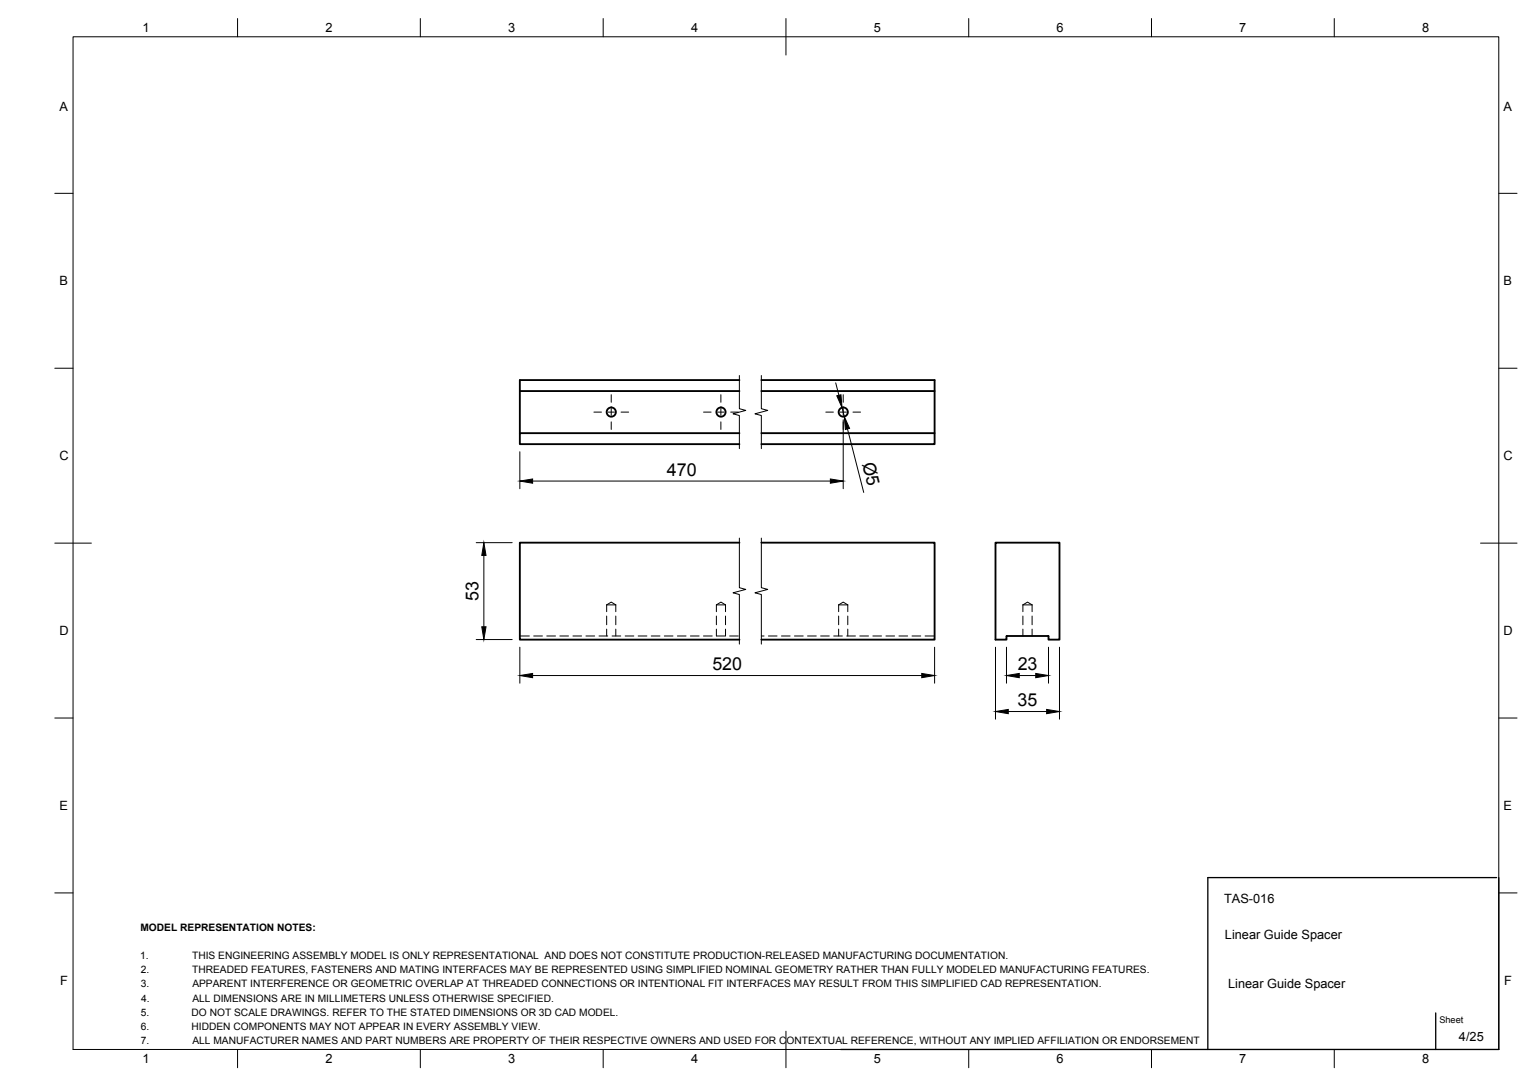
ISO-10303-21;
HEADER;
/* Generated by software containing ST-Developer
 * from STEP Tools, Inc. (www.steptools.com) 
 */

FILE_DESCRIPTION(
/* description */ ('STEP AP214'),
/* implementation_level */ '2;1');

FILE_NAME(
/* name */ 'Linear Guide Spacer.step',
/* time_stamp */ '2026-11-15T14:55:55-08:00',
/* author */ (''),
/* organization */ (''),
/* preprocessor_version */ 'ST-DEVELOPER v20.2',
/* originating_system */ 'Autodesk Translation Framework v15.17.0.0',
/* authorisation */ '');

FILE_SCHEMA (('AUTOMOTIVE_DESIGN { 1 0 10303 214 3 1 1 }'));
ENDSEC;

DATA;
#10=MECHANICAL_DESIGN_GEOMETRIC_PRESENTATION_REPRESENTATION('',(#953),#57079);
#891=SHAPE_REPRESENTATION_RELATIONSHIP('SRR','None',#57281,#920);
#920=ADVANCED_BREP_SHAPE_REPRESENTATION('',(#990),#57073);
#953=STYLED_ITEM('',(#57444),#990);
#990=MANIFOLD_SOLID_BREP('Body1',#24553);
#1318=FACE_BOUND('',#5120,.T.);
#1319=FACE_BOUND('',#5121,.T.);
#1320=FACE_BOUND('',#5122,.T.);
#1321=FACE_BOUND('',#5123,.T.);
#1322=FACE_BOUND('',#5124,.T.);
#1323=FACE_BOUND('',#5125,.T.);
#1324=FACE_BOUND('',#5126,.T.);
#1325=FACE_BOUND('',#5127,.T.);
#2021=PLANE('',#27222);
#2022=PLANE('',#27223);
#2023=PLANE('',#27226);
#2024=PLANE('',#27227);
#2025=PLANE('',#27230);
#2026=PLANE('',#27231);
#2027=PLANE('',#27232);
#2028=PLANE('',#27233);
#2029=PLANE('',#27234);
#2030=PLANE('',#27235);
#2141=CONICAL_SURFACE('',#27193,2.5,1.02974425867665);
#2142=CONICAL_SURFACE('',#27197,2.5,1.02974425867665);
#2143=CONICAL_SURFACE('',#27201,2.5,1.02974425867665);
#2144=CONICAL_SURFACE('',#27205,2.5,1.02974425867665);
#2145=CONICAL_SURFACE('',#27209,2.5,1.02974425867665);
#2146=CONICAL_SURFACE('',#27213,2.5,1.02974425867665);
#2147=CONICAL_SURFACE('',#27217,2.5,1.02974425867665);
#2148=CONICAL_SURFACE('',#27221,2.5,1.02974425867665);
#3402=FACE_OUTER_BOUND('',#5095,.T.);
#3403=FACE_OUTER_BOUND('',#5096,.T.);
#3404=FACE_OUTER_BOUND('',#5097,.T.);
#3405=FACE_OUTER_BOUND('',#5098,.T.);
#3406=FACE_OUTER_BOUND('',#5099,.T.);
#3407=FACE_OUTER_BOUND('',#5100,.T.);
#3408=FACE_OUTER_BOUND('',#5101,.T.);
#3409=FACE_OUTER_BOUND('',#5102,.T.);
#3410=FACE_OUTER_BOUND('',#5103,.T.);
#3411=FACE_OUTER_BOUND('',#5104,.T.);
#3412=FACE_OUTER_BOUND('',#5105,.T.);
#3413=FACE_OUTER_BOUND('',#5106,.T.);
#3414=FACE_OUTER_BOUND('',#5107,.T.);
#3415=FACE_OUTER_BOUND('',#5108,.T.);
#3416=FACE_OUTER_BOUND('',#5109,.T.);
#3417=FACE_OUTER_BOUND('',#5110,.T.);
#3418=FACE_OUTER_BOUND('',#5111,.T.);
#3419=FACE_OUTER_BOUND('',#5112,.T.);
#3420=FACE_OUTER_BOUND('',#5113,.T.);
#3421=FACE_OUTER_BOUND('',#5114,.T.);
#3422=FACE_OUTER_BOUND('',#5115,.T.);
#3423=FACE_OUTER_BOUND('',#5116,.T.);
#3424=FACE_OUTER_BOUND('',#5117,.T.);
#3425=FACE_OUTER_BOUND('',#5118,.T.);
#3426=FACE_OUTER_BOUND('',#5119,.T.);
#3427=FACE_OUTER_BOUND('',#5128,.T.);
#3428=FACE_OUTER_BOUND('',#5129,.T.);
#3429=FACE_OUTER_BOUND('',#5130,.T.);
#5095=EDGE_LOOP('',(#22196,#22197,#22198,#22199));
#5096=EDGE_LOOP('',(#22200,#22201,#22202));
#5097=EDGE_LOOP('',(#22203,#22204,#22205,#22206));
#5098=EDGE_LOOP('',(#22207,#22208,#22209));
#5099=EDGE_LOOP('',(#22210,#22211,#22212,#22213));
#5100=EDGE_LOOP('',(#22214,#22215,#22216));
#5101=EDGE_LOOP('',(#22217,#22218,#22219,#22220));
#5102=EDGE_LOOP('',(#22221,#22222,#22223));
#5103=EDGE_LOOP('',(#22224,#22225,#22226,#22227));
#5104=EDGE_LOOP('',(#22228,#22229,#22230));
#5105=EDGE_LOOP('',(#22231,#22232,#22233,#22234));
#5106=EDGE_LOOP('',(#22235,#22236,#22237));
#5107=EDGE_LOOP('',(#22238,#22239,#22240,#22241));
#5108=EDGE_LOOP('',(#22242,#22243,#22244));
#5109=EDGE_LOOP('',(#22245,#22246,#22247,#22248));
#5110=EDGE_LOOP('',(#22249,#22250,#22251));
#5111=EDGE_LOOP('',(#22252,#22253,#22254,#22255));
#5112=EDGE_LOOP('',(#22256,#22257,#22258,#22259,#22260,#22261,#22262,#22263,
#22264,#22265));
#5113=EDGE_LOOP('',(#22266,#22267,#22268,#22269));
#5114=EDGE_LOOP('',(#22270,#22271,#22272,#22273,#22274,#22275,#22276,#22277,
#22278,#22279));
#5115=EDGE_LOOP('',(#22280,#22281,#22282,#22283));
#5116=EDGE_LOOP('',(#22284,#22285,#22286,#22287));
#5117=EDGE_LOOP('',(#22288,#22289,#22290,#22291));
#5118=EDGE_LOOP('',(#22292,#22293,#22294,#22295));
#5119=EDGE_LOOP('',(#22296,#22297,#22298,#22299));
#5120=EDGE_LOOP('',(#22300));
#5121=EDGE_LOOP('',(#22301));
#5122=EDGE_LOOP('',(#22302));
#5123=EDGE_LOOP('',(#22303));
#5124=EDGE_LOOP('',(#22304));
#5125=EDGE_LOOP('',(#22305));
#5126=EDGE_LOOP('',(#22306));
#5127=EDGE_LOOP('',(#22307));
#5128=EDGE_LOOP('',(#22308,#22309,#22310,#22311));
#5129=EDGE_LOOP('',(#22312,#22313,#22314,#22315));
#5130=EDGE_LOOP('',(#22316,#22317,#22318,#22319));
#7032=LINE('',#56352,#8999);
#7033=LINE('',#56356,#9000);
#7034=LINE('',#56361,#9001);
#7035=LINE('',#56365,#9002);
#7036=LINE('',#56370,#9003);
#7037=LINE('',#56374,#9004);
#7038=LINE('',#56379,#9005);
#7039=LINE('',#56383,#9006);
#7040=LINE('',#56388,#9007);
#7041=LINE('',#56392,#9008);
#7042=LINE('',#56397,#9009);
#7043=LINE('',#56401,#9010);
#7044=LINE('',#56406,#9011);
#7045=LINE('',#56410,#9012);
#7046=LINE('',#56415,#9013);
#7047=LINE('',#56419,#9014);
#7048=LINE('',#56423,#9015);
#7049=LINE('',#56425,#9016);
#7050=LINE('',#56427,#9017);
#7051=LINE('',#56428,#9018);
#7052=LINE('',#56431,#9019);
#7053=LINE('',#56435,#9020);
#7054=LINE('',#56439,#9021);
#7055=LINE('',#56441,#9022);
#7056=LINE('',#56443,#9023);
#7057=LINE('',#56445,#9024);
#7058=LINE('',#56446,#9025);
#7059=LINE('',#56449,#9026);
#7060=LINE('',#56451,#9027);
#7061=LINE('',#56452,#9028);
#7062=LINE('',#56456,#9029);
#7063=LINE('',#56460,#9030);
#7064=LINE('',#56463,#9031);
#7065=LINE('',#56464,#9032);
#7066=LINE('',#56466,#9033);
#7067=LINE('',#56467,#9034);
#7068=LINE('',#56469,#9035);
#7069=LINE('',#56470,#9036);
#7070=LINE('',#56474,#9037);
#7071=LINE('',#56476,#9038);
#7072=LINE('',#56477,#9039);
#7073=LINE('',#56479,#9040);
#8999=VECTOR('',#33876,2.5);
#9000=VECTOR('',#33881,2.5);
#9001=VECTOR('',#33886,2.5);
#9002=VECTOR('',#33891,2.5);
#9003=VECTOR('',#33896,2.5);
#9004=VECTOR('',#33901,2.5);
#9005=VECTOR('',#33906,2.5);
#9006=VECTOR('',#33911,2.5);
#9007=VECTOR('',#33916,2.5);
#9008=VECTOR('',#33921,2.5);
#9009=VECTOR('',#33926,2.5);
#9010=VECTOR('',#33931,2.5);
#9011=VECTOR('',#33936,2.5);
#9012=VECTOR('',#33941,2.5);
#9013=VECTOR('',#33946,2.5);
#9014=VECTOR('',#33951,2.5);
#9015=VECTOR('',#33954,1000.);
#9016=VECTOR('',#33955,1000.);
#9017=VECTOR('',#33956,1000.);
#9018=VECTOR('',#33957,1000.);
#9019=VECTOR('',#33960,1000.);
#9020=VECTOR('',#33963,1000.);
#9021=VECTOR('',#33966,1000.);
#9022=VECTOR('',#33967,1000.);
#9023=VECTOR('',#33968,1000.);
#9024=VECTOR('',#33969,1000.);
#9025=VECTOR('',#33970,1000.);
#9026=VECTOR('',#33973,1000.);
#9027=VECTOR('',#33974,1000.);
#9028=VECTOR('',#33975,1000.);
#9029=VECTOR('',#33978,1000.);
#9030=VECTOR('',#33981,1000.);
#9031=VECTOR('',#33984,1000.);
#9032=VECTOR('',#33985,1000.);
#9033=VECTOR('',#33986,1000.);
#9034=VECTOR('',#33987,1000.);
#9035=VECTOR('',#33990,1000.);
#9036=VECTOR('',#33991,1000.);
#9037=VECTOR('',#33998,1000.);
#9038=VECTOR('',#34001,1000.);
#9039=VECTOR('',#34002,1000.);
#9040=VECTOR('',#34005,1000.);
#10192=CIRCLE('',#27191,2.5);
#10193=CIRCLE('',#27192,2.5);
#10194=CIRCLE('',#27195,2.5);
#10195=CIRCLE('',#27196,2.5);
#10196=CIRCLE('',#27199,2.5);
#10197=CIRCLE('',#27200,2.5);
#10198=CIRCLE('',#27203,2.5);
#10199=CIRCLE('',#27204,2.5);
#10200=CIRCLE('',#27207,2.5);
#10201=CIRCLE('',#27208,2.5);
#10202=CIRCLE('',#27211,2.5);
#10203=CIRCLE('',#27212,2.5);
#10204=CIRCLE('',#27215,2.5);
#10205=CIRCLE('',#27216,2.5);
#10206=CIRCLE('',#27219,2.5);
#10207=CIRCLE('',#27220,2.5);
#10208=CIRCLE('',#27224,0.200000000000001);
#10209=CIRCLE('',#27225,0.200000000000001);
#10210=CIRCLE('',#27228,0.200000000000001);
#10211=CIRCLE('',#27229,0.200000000000001);
#12322=VERTEX_POINT('',#56349);
#12323=VERTEX_POINT('',#56351);
#12324=VERTEX_POINT('',#56355);
#12325=VERTEX_POINT('',#56358);
#12326=VERTEX_POINT('',#56360);
#12327=VERTEX_POINT('',#56364);
#12328=VERTEX_POINT('',#56367);
#12329=VERTEX_POINT('',#56369);
#12330=VERTEX_POINT('',#56373);
#12331=VERTEX_POINT('',#56376);
#12332=VERTEX_POINT('',#56378);
#12333=VERTEX_POINT('',#56382);
#12334=VERTEX_POINT('',#56385);
#12335=VERTEX_POINT('',#56387);
#12336=VERTEX_POINT('',#56391);
#12337=VERTEX_POINT('',#56394);
#12338=VERTEX_POINT('',#56396);
#12339=VERTEX_POINT('',#56400);
#12340=VERTEX_POINT('',#56403);
#12341=VERTEX_POINT('',#56405);
#12342=VERTEX_POINT('',#56409);
#12343=VERTEX_POINT('',#56412);
#12344=VERTEX_POINT('',#56414);
#12345=VERTEX_POINT('',#56418);
#12346=VERTEX_POINT('',#56421);
#12347=VERTEX_POINT('',#56422);
#12348=VERTEX_POINT('',#56424);
#12349=VERTEX_POINT('',#56426);
#12350=VERTEX_POINT('',#56430);
#12351=VERTEX_POINT('',#56432);
#12352=VERTEX_POINT('',#56434);
#12353=VERTEX_POINT('',#56436);
#12354=VERTEX_POINT('',#56438);
#12355=VERTEX_POINT('',#56440);
#12356=VERTEX_POINT('',#56442);
#12357=VERTEX_POINT('',#56444);
#12358=VERTEX_POINT('',#56448);
#12359=VERTEX_POINT('',#56450);
#12360=VERTEX_POINT('',#56454);
#12361=VERTEX_POINT('',#56455);
#12362=VERTEX_POINT('',#56457);
#12363=VERTEX_POINT('',#56459);
#12364=VERTEX_POINT('',#56461);
#12365=VERTEX_POINT('',#56465);
#15643=EDGE_CURVE('',#12322,#12322,#10192,.T.);
#15644=EDGE_CURVE('',#12322,#12323,#7032,.T.);
#15645=EDGE_CURVE('',#12323,#12323,#10193,.T.);
#15646=EDGE_CURVE('',#12324,#12322,#7033,.T.);
#15647=EDGE_CURVE('',#12325,#12325,#10194,.T.);
#15648=EDGE_CURVE('',#12325,#12326,#7034,.T.);
#15649=EDGE_CURVE('',#12326,#12326,#10195,.T.);
#15650=EDGE_CURVE('',#12327,#12325,#7035,.T.);
#15651=EDGE_CURVE('',#12328,#12328,#10196,.T.);
#15652=EDGE_CURVE('',#12328,#12329,#7036,.T.);
#15653=EDGE_CURVE('',#12329,#12329,#10197,.T.);
#15654=EDGE_CURVE('',#12330,#12328,#7037,.T.);
#15655=EDGE_CURVE('',#12331,#12331,#10198,.T.);
#15656=EDGE_CURVE('',#12331,#12332,#7038,.T.);
#15657=EDGE_CURVE('',#12332,#12332,#10199,.T.);
#15658=EDGE_CURVE('',#12333,#12331,#7039,.T.);
#15659=EDGE_CURVE('',#12334,#12334,#10200,.T.);
#15660=EDGE_CURVE('',#12334,#12335,#7040,.T.);
#15661=EDGE_CURVE('',#12335,#12335,#10201,.T.);
#15662=EDGE_CURVE('',#12336,#12334,#7041,.T.);
#15663=EDGE_CURVE('',#12337,#12337,#10202,.T.);
#15664=EDGE_CURVE('',#12337,#12338,#7042,.T.);
#15665=EDGE_CURVE('',#12338,#12338,#10203,.T.);
#15666=EDGE_CURVE('',#12339,#12337,#7043,.T.);
#15667=EDGE_CURVE('',#12340,#12340,#10204,.T.);
#15668=EDGE_CURVE('',#12340,#12341,#7044,.T.);
#15669=EDGE_CURVE('',#12341,#12341,#10205,.T.);
#15670=EDGE_CURVE('',#12342,#12340,#7045,.T.);
#15671=EDGE_CURVE('',#12343,#12343,#10206,.T.);
#15672=EDGE_CURVE('',#12343,#12344,#7046,.T.);
#15673=EDGE_CURVE('',#12344,#12344,#10207,.T.);
#15674=EDGE_CURVE('',#12345,#12343,#7047,.T.);
#15675=EDGE_CURVE('',#12346,#12347,#7048,.T.);
#15676=EDGE_CURVE('',#12347,#12348,#7049,.T.);
#15677=EDGE_CURVE('',#12349,#12348,#7050,.T.);
#15678=EDGE_CURVE('',#12346,#12349,#7051,.T.);
#15679=EDGE_CURVE('',#12350,#12348,#7052,.T.);
#15680=EDGE_CURVE('',#12350,#12351,#10208,.T.);
#15681=EDGE_CURVE('',#12352,#12351,#7053,.T.);
#15682=EDGE_CURVE('',#12352,#12353,#10209,.T.);
#15683=EDGE_CURVE('',#12354,#12353,#7054,.T.);
#15684=EDGE_CURVE('',#12354,#12355,#7055,.T.);
#15685=EDGE_CURVE('',#12355,#12356,#7056,.T.);
#15686=EDGE_CURVE('',#12357,#12356,#7057,.T.);
#15687=EDGE_CURVE('',#12349,#12357,#7058,.T.);
#15688=EDGE_CURVE('',#12356,#12358,#7059,.T.);
#15689=EDGE_CURVE('',#12359,#12358,#7060,.T.);
#15690=EDGE_CURVE('',#12357,#12359,#7061,.T.);
#15691=EDGE_CURVE('',#12360,#12361,#7062,.T.);
#15692=EDGE_CURVE('',#12361,#12362,#10210,.T.);
#15693=EDGE_CURVE('',#12362,#12363,#7063,.T.);
#15694=EDGE_CURVE('',#12363,#12364,#10211,.T.);
#15695=EDGE_CURVE('',#12364,#12347,#7064,.T.);
#15696=EDGE_CURVE('',#12359,#12346,#7065,.T.);
#15697=EDGE_CURVE('',#12358,#12365,#7066,.T.);
#15698=EDGE_CURVE('',#12360,#12365,#7067,.T.);
#15699=EDGE_CURVE('',#12360,#12354,#7068,.T.);
#15700=EDGE_CURVE('',#12365,#12355,#7069,.T.);
#15701=EDGE_CURVE('',#12364,#12350,#7070,.T.);
#15702=EDGE_CURVE('',#12362,#12352,#7071,.T.);
#15703=EDGE_CURVE('',#12351,#12363,#7072,.T.);
#15704=EDGE_CURVE('',#12353,#12361,#7073,.T.);
#22196=ORIENTED_EDGE('',*,*,#15643,.F.);
#22197=ORIENTED_EDGE('',*,*,#15644,.T.);
#22198=ORIENTED_EDGE('',*,*,#15645,.T.);
#22199=ORIENTED_EDGE('',*,*,#15644,.F.);
#22200=ORIENTED_EDGE('',*,*,#15646,.T.);
#22201=ORIENTED_EDGE('',*,*,#15643,.T.);
#22202=ORIENTED_EDGE('',*,*,#15646,.F.);
#22203=ORIENTED_EDGE('',*,*,#15647,.F.);
#22204=ORIENTED_EDGE('',*,*,#15648,.T.);
#22205=ORIENTED_EDGE('',*,*,#15649,.T.);
#22206=ORIENTED_EDGE('',*,*,#15648,.F.);
#22207=ORIENTED_EDGE('',*,*,#15650,.T.);
#22208=ORIENTED_EDGE('',*,*,#15647,.T.);
#22209=ORIENTED_EDGE('',*,*,#15650,.F.);
#22210=ORIENTED_EDGE('',*,*,#15651,.F.);
#22211=ORIENTED_EDGE('',*,*,#15652,.T.);
#22212=ORIENTED_EDGE('',*,*,#15653,.T.);
#22213=ORIENTED_EDGE('',*,*,#15652,.F.);
#22214=ORIENTED_EDGE('',*,*,#15654,.T.);
#22215=ORIENTED_EDGE('',*,*,#15651,.T.);
#22216=ORIENTED_EDGE('',*,*,#15654,.F.);
#22217=ORIENTED_EDGE('',*,*,#15655,.F.);
#22218=ORIENTED_EDGE('',*,*,#15656,.T.);
#22219=ORIENTED_EDGE('',*,*,#15657,.T.);
#22220=ORIENTED_EDGE('',*,*,#15656,.F.);
#22221=ORIENTED_EDGE('',*,*,#15658,.T.);
#22222=ORIENTED_EDGE('',*,*,#15655,.T.);
#22223=ORIENTED_EDGE('',*,*,#15658,.F.);
#22224=ORIENTED_EDGE('',*,*,#15659,.F.);
#22225=ORIENTED_EDGE('',*,*,#15660,.T.);
#22226=ORIENTED_EDGE('',*,*,#15661,.T.);
#22227=ORIENTED_EDGE('',*,*,#15660,.F.);
#22228=ORIENTED_EDGE('',*,*,#15662,.T.);
#22229=ORIENTED_EDGE('',*,*,#15659,.T.);
#22230=ORIENTED_EDGE('',*,*,#15662,.F.);
#22231=ORIENTED_EDGE('',*,*,#15663,.F.);
#22232=ORIENTED_EDGE('',*,*,#15664,.T.);
#22233=ORIENTED_EDGE('',*,*,#15665,.T.);
#22234=ORIENTED_EDGE('',*,*,#15664,.F.);
#22235=ORIENTED_EDGE('',*,*,#15666,.T.);
#22236=ORIENTED_EDGE('',*,*,#15663,.T.);
#22237=ORIENTED_EDGE('',*,*,#15666,.F.);
#22238=ORIENTED_EDGE('',*,*,#15667,.F.);
#22239=ORIENTED_EDGE('',*,*,#15668,.T.);
#22240=ORIENTED_EDGE('',*,*,#15669,.T.);
#22241=ORIENTED_EDGE('',*,*,#15668,.F.);
#22242=ORIENTED_EDGE('',*,*,#15670,.T.);
#22243=ORIENTED_EDGE('',*,*,#15667,.T.);
#22244=ORIENTED_EDGE('',*,*,#15670,.F.);
#22245=ORIENTED_EDGE('',*,*,#15671,.F.);
#22246=ORIENTED_EDGE('',*,*,#15672,.T.);
#22247=ORIENTED_EDGE('',*,*,#15673,.T.);
#22248=ORIENTED_EDGE('',*,*,#15672,.F.);
#22249=ORIENTED_EDGE('',*,*,#15674,.T.);
#22250=ORIENTED_EDGE('',*,*,#15671,.T.);
#22251=ORIENTED_EDGE('',*,*,#15674,.F.);
#22252=ORIENTED_EDGE('',*,*,#15675,.T.);
#22253=ORIENTED_EDGE('',*,*,#15676,.T.);
#22254=ORIENTED_EDGE('',*,*,#15677,.F.);
#22255=ORIENTED_EDGE('',*,*,#15678,.F.);
#22256=ORIENTED_EDGE('',*,*,#15677,.T.);
#22257=ORIENTED_EDGE('',*,*,#15679,.F.);
#22258=ORIENTED_EDGE('',*,*,#15680,.T.);
#22259=ORIENTED_EDGE('',*,*,#15681,.F.);
#22260=ORIENTED_EDGE('',*,*,#15682,.T.);
#22261=ORIENTED_EDGE('',*,*,#15683,.F.);
#22262=ORIENTED_EDGE('',*,*,#15684,.T.);
#22263=ORIENTED_EDGE('',*,*,#15685,.T.);
#22264=ORIENTED_EDGE('',*,*,#15686,.F.);
#22265=ORIENTED_EDGE('',*,*,#15687,.F.);
#22266=ORIENTED_EDGE('',*,*,#15688,.T.);
#22267=ORIENTED_EDGE('',*,*,#15689,.F.);
#22268=ORIENTED_EDGE('',*,*,#15690,.F.);
#22269=ORIENTED_EDGE('',*,*,#15686,.T.);
#22270=ORIENTED_EDGE('',*,*,#15691,.T.);
#22271=ORIENTED_EDGE('',*,*,#15692,.T.);
#22272=ORIENTED_EDGE('',*,*,#15693,.T.);
#22273=ORIENTED_EDGE('',*,*,#15694,.T.);
#22274=ORIENTED_EDGE('',*,*,#15695,.T.);
#22275=ORIENTED_EDGE('',*,*,#15675,.F.);
#22276=ORIENTED_EDGE('',*,*,#15696,.F.);
#22277=ORIENTED_EDGE('',*,*,#15689,.T.);
#22278=ORIENTED_EDGE('',*,*,#15697,.T.);
#22279=ORIENTED_EDGE('',*,*,#15698,.F.);
#22280=ORIENTED_EDGE('',*,*,#15684,.F.);
#22281=ORIENTED_EDGE('',*,*,#15699,.F.);
#22282=ORIENTED_EDGE('',*,*,#15698,.T.);
#22283=ORIENTED_EDGE('',*,*,#15700,.T.);
#22284=ORIENTED_EDGE('',*,*,#15687,.T.);
#22285=ORIENTED_EDGE('',*,*,#15690,.T.);
#22286=ORIENTED_EDGE('',*,*,#15696,.T.);
#22287=ORIENTED_EDGE('',*,*,#15678,.T.);
#22288=ORIENTED_EDGE('',*,*,#15685,.F.);
#22289=ORIENTED_EDGE('',*,*,#15700,.F.);
#22290=ORIENTED_EDGE('',*,*,#15697,.F.);
#22291=ORIENTED_EDGE('',*,*,#15688,.F.);
#22292=ORIENTED_EDGE('',*,*,#15695,.F.);
#22293=ORIENTED_EDGE('',*,*,#15701,.T.);
#22294=ORIENTED_EDGE('',*,*,#15679,.T.);
#22295=ORIENTED_EDGE('',*,*,#15676,.F.);
#22296=ORIENTED_EDGE('',*,*,#15693,.F.);
#22297=ORIENTED_EDGE('',*,*,#15702,.T.);
#22298=ORIENTED_EDGE('',*,*,#15681,.T.);
#22299=ORIENTED_EDGE('',*,*,#15703,.T.);
#22300=ORIENTED_EDGE('',*,*,#15645,.F.);
#22301=ORIENTED_EDGE('',*,*,#15649,.F.);
#22302=ORIENTED_EDGE('',*,*,#15653,.F.);
#22303=ORIENTED_EDGE('',*,*,#15657,.F.);
#22304=ORIENTED_EDGE('',*,*,#15661,.F.);
#22305=ORIENTED_EDGE('',*,*,#15665,.F.);
#22306=ORIENTED_EDGE('',*,*,#15669,.F.);
#22307=ORIENTED_EDGE('',*,*,#15673,.F.);
#22308=ORIENTED_EDGE('',*,*,#15683,.T.);
#22309=ORIENTED_EDGE('',*,*,#15704,.T.);
#22310=ORIENTED_EDGE('',*,*,#15691,.F.);
#22311=ORIENTED_EDGE('',*,*,#15699,.T.);
#22312=ORIENTED_EDGE('',*,*,#15692,.F.);
#22313=ORIENTED_EDGE('',*,*,#15704,.F.);
#22314=ORIENTED_EDGE('',*,*,#15682,.F.);
#22315=ORIENTED_EDGE('',*,*,#15702,.F.);
#22316=ORIENTED_EDGE('',*,*,#15694,.F.);
#22317=ORIENTED_EDGE('',*,*,#15703,.F.);
#22318=ORIENTED_EDGE('',*,*,#15680,.F.);
#22319=ORIENTED_EDGE('',*,*,#15701,.F.);
#23121=CYLINDRICAL_SURFACE('',#27190,2.5);
#23122=CYLINDRICAL_SURFACE('',#27194,2.5);
#23123=CYLINDRICAL_SURFACE('',#27198,2.5);
#23124=CYLINDRICAL_SURFACE('',#27202,2.5);
#23125=CYLINDRICAL_SURFACE('',#27206,2.5);
#23126=CYLINDRICAL_SURFACE('',#27210,2.5);
#23127=CYLINDRICAL_SURFACE('',#27214,2.5);
#23128=CYLINDRICAL_SURFACE('',#27218,2.5);
#23129=CYLINDRICAL_SURFACE('',#27236,0.200000000000001);
#23130=CYLINDRICAL_SURFACE('',#27237,0.200000000000001);
#24394=ADVANCED_FACE('',(#3402),#23121,.F.);
#24395=ADVANCED_FACE('',(#3403),#2141,.F.);
#24396=ADVANCED_FACE('',(#3404),#23122,.F.);
#24397=ADVANCED_FACE('',(#3405),#2142,.F.);
#24398=ADVANCED_FACE('',(#3406),#23123,.F.);
#24399=ADVANCED_FACE('',(#3407),#2143,.F.);
#24400=ADVANCED_FACE('',(#3408),#23124,.F.);
#24401=ADVANCED_FACE('',(#3409),#2144,.F.);
#24402=ADVANCED_FACE('',(#3410),#23125,.F.);
#24403=ADVANCED_FACE('',(#3411),#2145,.F.);
#24404=ADVANCED_FACE('',(#3412),#23126,.F.);
#24405=ADVANCED_FACE('',(#3413),#2146,.F.);
#24406=ADVANCED_FACE('',(#3414),#23127,.F.);
#24407=ADVANCED_FACE('',(#3415),#2147,.F.);
#24408=ADVANCED_FACE('',(#3416),#23128,.F.);
#24409=ADVANCED_FACE('',(#3417),#2148,.F.);
#24410=ADVANCED_FACE('',(#3418),#2021,.F.);
#24411=ADVANCED_FACE('',(#3419),#2022,.F.);
#24412=ADVANCED_FACE('',(#3420),#2023,.F.);
#24413=ADVANCED_FACE('',(#3421),#2024,.F.);
#24414=ADVANCED_FACE('',(#3422),#2025,.F.);
#24415=ADVANCED_FACE('',(#3423),#2026,.T.);
#24416=ADVANCED_FACE('',(#3424),#2027,.F.);
#24417=ADVANCED_FACE('',(#3425),#2028,.F.);
#24418=ADVANCED_FACE('',(#3426,#1318,#1319,#1320,#1321,#1322,#1323,#1324,
#1325),#2029,.F.);
#24419=ADVANCED_FACE('',(#3427),#2030,.F.);
#24420=ADVANCED_FACE('',(#3428),#23129,.F.);
#24421=ADVANCED_FACE('',(#3429),#23130,.F.);
#24553=CLOSED_SHELL('',(#24394,#24395,#24396,#24397,#24398,#24399,#24400,
#24401,#24402,#24403,#24404,#24405,#24406,#24407,#24408,#24409,#24410,#24411,
#24412,#24413,#24414,#24415,#24416,#24417,#24418,#24419,#24420,#24421));
#27189=AXIS2_PLACEMENT_3D('',#56347,#33870,#33871);
#27190=AXIS2_PLACEMENT_3D('',#56348,#33872,#33873);
#27191=AXIS2_PLACEMENT_3D('',#56350,#33874,#33875);
#27192=AXIS2_PLACEMENT_3D('',#56353,#33877,#33878);
#27193=AXIS2_PLACEMENT_3D('',#56354,#33879,#33880);
#27194=AXIS2_PLACEMENT_3D('',#56357,#33882,#33883);
#27195=AXIS2_PLACEMENT_3D('',#56359,#33884,#33885);
#27196=AXIS2_PLACEMENT_3D('',#56362,#33887,#33888);
#27197=AXIS2_PLACEMENT_3D('',#56363,#33889,#33890);
#27198=AXIS2_PLACEMENT_3D('',#56366,#33892,#33893);
#27199=AXIS2_PLACEMENT_3D('',#56368,#33894,#33895);
#27200=AXIS2_PLACEMENT_3D('',#56371,#33897,#33898);
#27201=AXIS2_PLACEMENT_3D('',#56372,#33899,#33900);
#27202=AXIS2_PLACEMENT_3D('',#56375,#33902,#33903);
#27203=AXIS2_PLACEMENT_3D('',#56377,#33904,#33905);
#27204=AXIS2_PLACEMENT_3D('',#56380,#33907,#33908);
#27205=AXIS2_PLACEMENT_3D('',#56381,#33909,#33910);
#27206=AXIS2_PLACEMENT_3D('',#56384,#33912,#33913);
#27207=AXIS2_PLACEMENT_3D('',#56386,#33914,#33915);
#27208=AXIS2_PLACEMENT_3D('',#56389,#33917,#33918);
#27209=AXIS2_PLACEMENT_3D('',#56390,#33919,#33920);
#27210=AXIS2_PLACEMENT_3D('',#56393,#33922,#33923);
#27211=AXIS2_PLACEMENT_3D('',#56395,#33924,#33925);
#27212=AXIS2_PLACEMENT_3D('',#56398,#33927,#33928);
#27213=AXIS2_PLACEMENT_3D('',#56399,#33929,#33930);
#27214=AXIS2_PLACEMENT_3D('',#56402,#33932,#33933);
#27215=AXIS2_PLACEMENT_3D('',#56404,#33934,#33935);
#27216=AXIS2_PLACEMENT_3D('',#56407,#33937,#33938);
#27217=AXIS2_PLACEMENT_3D('',#56408,#33939,#33940);
#27218=AXIS2_PLACEMENT_3D('',#56411,#33942,#33943);
#27219=AXIS2_PLACEMENT_3D('',#56413,#33944,#33945);
#27220=AXIS2_PLACEMENT_3D('',#56416,#33947,#33948);
#27221=AXIS2_PLACEMENT_3D('',#56417,#33949,#33950);
#27222=AXIS2_PLACEMENT_3D('',#56420,#33952,#33953);
#27223=AXIS2_PLACEMENT_3D('',#56429,#33958,#33959);
#27224=AXIS2_PLACEMENT_3D('',#56433,#33961,#33962);
#27225=AXIS2_PLACEMENT_3D('',#56437,#33964,#33965);
#27226=AXIS2_PLACEMENT_3D('',#56447,#33971,#33972);
#27227=AXIS2_PLACEMENT_3D('',#56453,#33976,#33977);
#27228=AXIS2_PLACEMENT_3D('',#56458,#33979,#33980);
#27229=AXIS2_PLACEMENT_3D('',#56462,#33982,#33983);
#27230=AXIS2_PLACEMENT_3D('',#56468,#33988,#33989);
#27231=AXIS2_PLACEMENT_3D('',#56471,#33992,#33993);
#27232=AXIS2_PLACEMENT_3D('',#56472,#33994,#33995);
#27233=AXIS2_PLACEMENT_3D('',#56473,#33996,#33997);
#27234=AXIS2_PLACEMENT_3D('',#56475,#33999,#34000);
#27235=AXIS2_PLACEMENT_3D('',#56478,#34003,#34004);
#27236=AXIS2_PLACEMENT_3D('',#56480,#34006,#34007);
#27237=AXIS2_PLACEMENT_3D('',#56481,#34008,#34009);
#33870=DIRECTION('axis',(0.,0.,1.));
#33871=DIRECTION('refdir',(1.,0.,0.));
#33872=DIRECTION('center_axis',(0.,-1.,0.));
#33873=DIRECTION('ref_axis',(0.,0.,-1.));
#33874=DIRECTION('center_axis',(0.,-1.,0.));
#33875=DIRECTION('ref_axis',(0.,0.,-1.));
#33876=DIRECTION('',(0.,-1.,0.));
#33877=DIRECTION('center_axis',(0.,-1.,0.));
#33878=DIRECTION('ref_axis',(0.,0.,-1.));
#33879=DIRECTION('center_axis',(0.,-1.,0.));
#33880=DIRECTION('ref_axis',(0.,0.,-1.));
#33881=DIRECTION('',(-1.04972719113862E-16,-0.515038074910054,0.857167300702112));
#33882=DIRECTION('center_axis',(0.,-1.,0.));
#33883=DIRECTION('ref_axis',(0.,0.,-1.));
#33884=DIRECTION('center_axis',(0.,-1.,0.));
#33885=DIRECTION('ref_axis',(0.,0.,-1.));
#33886=DIRECTION('',(0.,-1.,0.));
#33887=DIRECTION('center_axis',(0.,-1.,0.));
#33888=DIRECTION('ref_axis',(0.,0.,-1.));
#33889=DIRECTION('center_axis',(0.,-1.,0.));
#33890=DIRECTION('ref_axis',(0.,0.,-1.));
#33891=DIRECTION('',(-1.04972719113862E-16,-0.515038074910054,0.857167300702112));
#33892=DIRECTION('center_axis',(0.,-1.,0.));
#33893=DIRECTION('ref_axis',(0.,0.,-1.));
#33894=DIRECTION('center_axis',(0.,-1.,0.));
#33895=DIRECTION('ref_axis',(0.,0.,-1.));
#33896=DIRECTION('',(0.,-1.,0.));
#33897=DIRECTION('center_axis',(0.,-1.,0.));
#33898=DIRECTION('ref_axis',(0.,0.,-1.));
#33899=DIRECTION('center_axis',(0.,-1.,0.));
#33900=DIRECTION('ref_axis',(0.,0.,-1.));
#33901=DIRECTION('',(-1.04972719113862E-16,-0.515038074910054,0.857167300702112));
#33902=DIRECTION('center_axis',(0.,-1.,0.));
#33903=DIRECTION('ref_axis',(0.,0.,-1.));
#33904=DIRECTION('center_axis',(0.,-1.,0.));
#33905=DIRECTION('ref_axis',(0.,0.,-1.));
#33906=DIRECTION('',(0.,-1.,0.));
#33907=DIRECTION('center_axis',(0.,-1.,0.));
#33908=DIRECTION('ref_axis',(0.,0.,-1.));
#33909=DIRECTION('center_axis',(0.,-1.,0.));
#33910=DIRECTION('ref_axis',(0.,0.,-1.));
#33911=DIRECTION('',(-1.04972719113862E-16,-0.515038074910056,0.857167300702111));
#33912=DIRECTION('center_axis',(0.,-1.,0.));
#33913=DIRECTION('ref_axis',(0.,0.,-1.));
#33914=DIRECTION('center_axis',(0.,-1.,0.));
#33915=DIRECTION('ref_axis',(0.,0.,-1.));
#33916=DIRECTION('',(0.,-1.,0.));
#33917=DIRECTION('center_axis',(0.,-1.,0.));
#33918=DIRECTION('ref_axis',(0.,0.,-1.));
#33919=DIRECTION('center_axis',(0.,-1.,0.));
#33920=DIRECTION('ref_axis',(0.,0.,-1.));
#33921=DIRECTION('',(-1.04972719113862E-16,-0.515038074910056,0.857167300702111));
#33922=DIRECTION('center_axis',(0.,-1.,0.));
#33923=DIRECTION('ref_axis',(0.,0.,-1.));
#33924=DIRECTION('center_axis',(0.,-1.,0.));
#33925=DIRECTION('ref_axis',(0.,0.,-1.));
#33926=DIRECTION('',(0.,-1.,0.));
#33927=DIRECTION('center_axis',(0.,-1.,0.));
#33928=DIRECTION('ref_axis',(0.,0.,-1.));
#33929=DIRECTION('center_axis',(0.,-1.,0.));
#33930=DIRECTION('ref_axis',(0.,0.,-1.));
#33931=DIRECTION('',(-1.04972719113862E-16,-0.515038074910054,0.857167300702112));
#33932=DIRECTION('center_axis',(0.,-1.,0.));
#33933=DIRECTION('ref_axis',(0.,0.,-1.));
#33934=DIRECTION('center_axis',(0.,-1.,0.));
#33935=DIRECTION('ref_axis',(0.,0.,-1.));
#33936=DIRECTION('',(0.,-1.,0.));
#33937=DIRECTION('center_axis',(0.,-1.,0.));
#33938=DIRECTION('ref_axis',(0.,0.,-1.));
#33939=DIRECTION('center_axis',(0.,-1.,0.));
#33940=DIRECTION('ref_axis',(0.,0.,-1.));
#33941=DIRECTION('',(-1.04972719113862E-16,-0.515038074910054,0.857167300702112));
#33942=DIRECTION('center_axis',(0.,-1.,0.));
#33943=DIRECTION('ref_axis',(0.,0.,-1.));
#33944=DIRECTION('center_axis',(0.,-1.,0.));
#33945=DIRECTION('ref_axis',(0.,0.,-1.));
#33946=DIRECTION('',(0.,-1.,0.));
#33947=DIRECTION('center_axis',(0.,-1.,0.));
#33948=DIRECTION('ref_axis',(0.,0.,-1.));
#33949=DIRECTION('center_axis',(0.,-1.,0.));
#33950=DIRECTION('ref_axis',(0.,0.,-1.));
#33951=DIRECTION('',(-1.04972719113862E-16,-0.515038074910054,0.857167300702112));
#33952=DIRECTION('center_axis',(0.,1.,0.));
#33953=DIRECTION('ref_axis',(0.,0.,1.));
#33954=DIRECTION('',(0.,0.,-1.));
#33955=DIRECTION('',(1.,0.,0.));
#33956=DIRECTION('',(0.,0.,-1.));
#33957=DIRECTION('',(1.,0.,0.));
#33958=DIRECTION('center_axis',(-1.,0.,0.));
#33959=DIRECTION('ref_axis',(0.,0.,1.));
#33960=DIRECTION('',(0.,-1.,0.));
#33961=DIRECTION('center_axis',(-1.,0.,0.));
#33962=DIRECTION('ref_axis',(0.,0.,1.));
#33963=DIRECTION('',(0.,0.,1.));
#33964=DIRECTION('center_axis',(-1.,0.,0.));
#33965=DIRECTION('ref_axis',(0.,0.,1.));
#33966=DIRECTION('',(0.,1.,0.));
#33967=DIRECTION('',(0.,0.,-1.));
#33968=DIRECTION('',(0.,1.,0.));
#33969=DIRECTION('',(0.,0.,-1.));
#33970=DIRECTION('',(0.,1.,0.));
#33971=DIRECTION('center_axis',(0.,-1.,0.));
#33972=DIRECTION('ref_axis',(0.,0.,-1.));
#33973=DIRECTION('',(-1.,0.,0.));
#33974=DIRECTION('',(0.,0.,-1.));
#33975=DIRECTION('',(-1.,0.,0.));
#33976=DIRECTION('center_axis',(1.,0.,0.));
#33977=DIRECTION('ref_axis',(0.,0.,-1.));
#33978=DIRECTION('',(0.,1.,0.));
#33979=DIRECTION('center_axis',(1.,0.,0.));
#33980=DIRECTION('ref_axis',(0.,0.,-1.));
#33981=DIRECTION('',(0.,0.,1.));
#33982=DIRECTION('center_axis',(1.,0.,0.));
#33983=DIRECTION('ref_axis',(0.,0.,-1.));
#33984=DIRECTION('',(0.,-1.,0.));
#33985=DIRECTION('',(0.,-1.,0.));
#33986=DIRECTION('',(0.,-1.,0.));
#33987=DIRECTION('',(0.,0.,-1.));
#33988=DIRECTION('center_axis',(0.,1.,0.));
#33989=DIRECTION('ref_axis',(0.,0.,1.));
#33990=DIRECTION('',(1.,0.,0.));
#33991=DIRECTION('',(1.,0.,0.));
#33992=DIRECTION('center_axis',(0.,0.,1.));
#33993=DIRECTION('ref_axis',(1.,0.,0.));
#33994=DIRECTION('center_axis',(0.,0.,1.));
#33995=DIRECTION('ref_axis',(1.,0.,0.));
#33996=DIRECTION('center_axis',(0.,0.,1.));
#33997=DIRECTION('ref_axis',(1.,0.,0.));
#33998=DIRECTION('',(1.,0.,0.));
#33999=DIRECTION('center_axis',(0.,1.,0.));
#34000=DIRECTION('ref_axis',(0.,0.,1.));
#34001=DIRECTION('',(1.,0.,0.));
#34002=DIRECTION('',(-1.,0.,0.));
#34003=DIRECTION('center_axis',(0.,0.,-1.));
#34004=DIRECTION('ref_axis',(-1.,0.,0.));
#34005=DIRECTION('',(-1.,0.,0.));
#34006=DIRECTION('center_axis',(-1.,0.,0.));
#34007=DIRECTION('ref_axis',(0.,0.,1.));
#34008=DIRECTION('center_axis',(-1.,0.,0.));
#34009=DIRECTION('ref_axis',(0.,0.,1.));
#56347=CARTESIAN_POINT('',(0.,0.,0.));
#56348=CARTESIAN_POINT('Origin',(-210.,-24.5,0.));
#56349=CARTESIAN_POINT('',(-210.,-7.49999999999999,2.5));
#56350=CARTESIAN_POINT('Origin',(-210.,-7.49999999999999,0.));
#56351=CARTESIAN_POINT('',(-210.,-24.5,2.5));
#56352=CARTESIAN_POINT('',(-210.,-24.5,2.5));
#56353=CARTESIAN_POINT('Origin',(-210.,-24.5,0.));
#56354=CARTESIAN_POINT('Origin',(-210.,-7.49999999999999,0.));
#56355=CARTESIAN_POINT('',(-210.,-5.99784845243109,0.));
#56356=CARTESIAN_POINT('',(-210.,-7.49999999999999,2.5));
#56357=CARTESIAN_POINT('Origin',(-150.,-24.5,0.));
#56358=CARTESIAN_POINT('',(-150.,-7.49999999999999,2.5));
#56359=CARTESIAN_POINT('Origin',(-150.,-7.49999999999999,0.));
#56360=CARTESIAN_POINT('',(-150.,-24.5,2.5));
#56361=CARTESIAN_POINT('',(-150.,-24.5,2.5));
#56362=CARTESIAN_POINT('Origin',(-150.,-24.5,0.));
#56363=CARTESIAN_POINT('Origin',(-150.,-7.49999999999999,0.));
#56364=CARTESIAN_POINT('',(-150.,-5.99784845243109,0.));
#56365=CARTESIAN_POINT('',(-150.,-7.49999999999999,2.5));
#56366=CARTESIAN_POINT('Origin',(-89.9999999999999,-24.5,0.));
#56367=CARTESIAN_POINT('',(-89.9999999999999,-7.49999999999999,2.5));
#56368=CARTESIAN_POINT('Origin',(-89.9999999999999,-7.49999999999999,0.));
#56369=CARTESIAN_POINT('',(-89.9999999999999,-24.5,2.5));
#56370=CARTESIAN_POINT('',(-89.9999999999999,-24.5,2.5));
#56371=CARTESIAN_POINT('Origin',(-89.9999999999999,-24.5,0.));
#56372=CARTESIAN_POINT('Origin',(-89.9999999999999,-7.49999999999999,0.));
#56373=CARTESIAN_POINT('',(-89.9999999999999,-5.99784845243109,0.));
#56374=CARTESIAN_POINT('',(-89.9999999999999,-7.49999999999999,2.5));
#56375=CARTESIAN_POINT('Origin',(-29.9999999999999,-24.5,0.));
#56376=CARTESIAN_POINT('',(-29.9999999999999,-7.49999999999999,2.5));
#56377=CARTESIAN_POINT('Origin',(-29.9999999999999,-7.49999999999999,0.));
#56378=CARTESIAN_POINT('',(-29.9999999999999,-24.5,2.5));
#56379=CARTESIAN_POINT('',(-29.9999999999999,-24.5,2.5));
#56380=CARTESIAN_POINT('Origin',(-29.9999999999999,-24.5,0.));
#56381=CARTESIAN_POINT('Origin',(-29.9999999999999,-7.49999999999999,0.));
#56382=CARTESIAN_POINT('',(-29.9999999999999,-5.99784845243109,0.));
#56383=CARTESIAN_POINT('',(-29.9999999999999,-7.49999999999999,2.5));
#56384=CARTESIAN_POINT('Origin',(30.0000000000001,-24.5,0.));
#56385=CARTESIAN_POINT('',(30.0000000000001,-7.49999999999999,2.5));
#56386=CARTESIAN_POINT('Origin',(30.0000000000001,-7.49999999999999,0.));
#56387=CARTESIAN_POINT('',(30.0000000000001,-24.5,2.5));
#56388=CARTESIAN_POINT('',(30.0000000000001,-24.5,2.5));
#56389=CARTESIAN_POINT('Origin',(30.0000000000001,-24.5,0.));
#56390=CARTESIAN_POINT('Origin',(30.0000000000001,-7.49999999999999,0.));
#56391=CARTESIAN_POINT('',(30.0000000000001,-5.99784845243109,0.));
#56392=CARTESIAN_POINT('',(30.0000000000001,-7.49999999999999,2.5));
#56393=CARTESIAN_POINT('Origin',(90.0000000000001,-24.5,0.));
#56394=CARTESIAN_POINT('',(90.0000000000001,-7.49999999999999,2.5));
#56395=CARTESIAN_POINT('Origin',(90.0000000000001,-7.49999999999999,0.));
#56396=CARTESIAN_POINT('',(90.0000000000001,-24.5,2.5));
#56397=CARTESIAN_POINT('',(90.0000000000001,-24.5,2.5));
#56398=CARTESIAN_POINT('Origin',(90.0000000000001,-24.5,0.));
#56399=CARTESIAN_POINT('Origin',(90.0000000000001,-7.49999999999999,0.));
#56400=CARTESIAN_POINT('',(90.0000000000001,-5.99784845243109,0.));
#56401=CARTESIAN_POINT('',(90.0000000000001,-7.49999999999999,2.5));
#56402=CARTESIAN_POINT('Origin',(150.,-24.5,0.));
#56403=CARTESIAN_POINT('',(150.,-7.49999999999999,2.5));
#56404=CARTESIAN_POINT('Origin',(150.,-7.49999999999999,0.));
#56405=CARTESIAN_POINT('',(150.,-24.5,2.5));
#56406=CARTESIAN_POINT('',(150.,-24.5,2.5));
#56407=CARTESIAN_POINT('Origin',(150.,-24.5,0.));
#56408=CARTESIAN_POINT('Origin',(150.,-7.49999999999999,0.));
#56409=CARTESIAN_POINT('',(150.,-5.99784845243109,0.));
#56410=CARTESIAN_POINT('',(150.,-7.49999999999999,2.5));
#56411=CARTESIAN_POINT('Origin',(210.,-24.5,0.));
#56412=CARTESIAN_POINT('',(210.,-7.49999999999999,2.5));
#56413=CARTESIAN_POINT('Origin',(210.,-7.49999999999999,0.));
#56414=CARTESIAN_POINT('',(210.,-24.5,2.5));
#56415=CARTESIAN_POINT('',(210.,-24.5,2.5));
#56416=CARTESIAN_POINT('Origin',(210.,-24.5,0.));
#56417=CARTESIAN_POINT('Origin',(210.,-7.49999999999999,0.));
#56418=CARTESIAN_POINT('',(210.,-5.99784845243109,0.));
#56419=CARTESIAN_POINT('',(210.,-7.49999999999999,2.5));
#56420=CARTESIAN_POINT('Origin',(-260.,-26.5,17.5));
#56421=CARTESIAN_POINT('',(-260.,-26.5,17.5));
#56422=CARTESIAN_POINT('',(-260.,-26.5,11.5));
#56423=CARTESIAN_POINT('',(-260.,-26.5,17.5));
#56424=CARTESIAN_POINT('',(260.,-26.5,11.5));
#56425=CARTESIAN_POINT('',(-260.,-26.5,11.5));
#56426=CARTESIAN_POINT('',(260.,-26.5,17.5));
#56427=CARTESIAN_POINT('',(260.,-26.5,17.5));
#56428=CARTESIAN_POINT('',(-260.,-26.5,17.5));
#56429=CARTESIAN_POINT('Origin',(260.,26.5,17.5));
#56430=CARTESIAN_POINT('',(260.,-24.7,11.5));
#56431=CARTESIAN_POINT('',(260.,-26.5,11.5));
#56432=CARTESIAN_POINT('',(260.,-24.5,11.3));
#56433=CARTESIAN_POINT('Origin',(260.,-24.7,11.3));
#56434=CARTESIAN_POINT('',(260.,-24.5,-11.3));
#56435=CARTESIAN_POINT('',(260.,-24.5,11.5));
#56436=CARTESIAN_POINT('',(260.,-24.7,-11.5));
#56437=CARTESIAN_POINT('Origin',(260.,-24.7,-11.3));
#56438=CARTESIAN_POINT('',(260.,-26.5,-11.5));
#56439=CARTESIAN_POINT('',(260.,-26.5,-11.5));
#56440=CARTESIAN_POINT('',(260.,-26.5,-17.5));
#56441=CARTESIAN_POINT('',(260.,-26.5,17.5));
#56442=CARTESIAN_POINT('',(260.,26.5,-17.5));
#56443=CARTESIAN_POINT('',(260.,26.5,-17.5));
#56444=CARTESIAN_POINT('',(260.,26.5,17.5));
#56445=CARTESIAN_POINT('',(260.,26.5,17.5));
#56446=CARTESIAN_POINT('',(260.,26.5,17.5));
#56447=CARTESIAN_POINT('Origin',(-260.,26.5,17.5));
#56448=CARTESIAN_POINT('',(-260.,26.5,-17.5));
#56449=CARTESIAN_POINT('',(-260.,26.5,-17.5));
#56450=CARTESIAN_POINT('',(-260.,26.5,17.5));
#56451=CARTESIAN_POINT('',(-260.,26.5,17.5));
#56452=CARTESIAN_POINT('',(-260.,26.5,17.5));
#56453=CARTESIAN_POINT('Origin',(-260.,26.5,17.5));
#56454=CARTESIAN_POINT('',(-260.,-26.5,-11.5));
#56455=CARTESIAN_POINT('',(-260.,-24.7,-11.5));
#56456=CARTESIAN_POINT('',(-260.,-26.5,-11.5));
#56457=CARTESIAN_POINT('',(-260.,-24.5,-11.3));
#56458=CARTESIAN_POINT('Origin',(-260.,-24.7,-11.3));
#56459=CARTESIAN_POINT('',(-260.,-24.5,11.3));
#56460=CARTESIAN_POINT('',(-260.,-24.5,11.5));
#56461=CARTESIAN_POINT('',(-260.,-24.7,11.5));
#56462=CARTESIAN_POINT('Origin',(-260.,-24.7,11.3));
#56463=CARTESIAN_POINT('',(-260.,-26.5,11.5));
#56464=CARTESIAN_POINT('',(-260.,26.5,17.5));
#56465=CARTESIAN_POINT('',(-260.,-26.5,-17.5));
#56466=CARTESIAN_POINT('',(-260.,26.5,-17.5));
#56467=CARTESIAN_POINT('',(-260.,-26.5,17.5));
#56468=CARTESIAN_POINT('Origin',(-260.,-26.5,17.5));
#56469=CARTESIAN_POINT('',(-260.,-26.5,-11.5));
#56470=CARTESIAN_POINT('',(-260.,-26.5,-17.5));
#56471=CARTESIAN_POINT('Origin',(0.,0.,17.5));
#56472=CARTESIAN_POINT('Origin',(0.,0.,-17.5));
#56473=CARTESIAN_POINT('Origin',(-260.,-26.5,11.5));
#56474=CARTESIAN_POINT('',(260.,-24.7,11.5));
#56475=CARTESIAN_POINT('Origin',(-260.,-24.5,11.5));
#56476=CARTESIAN_POINT('',(260.,-24.5,-11.3));
#56477=CARTESIAN_POINT('',(-260.,-24.5,11.3));
#56478=CARTESIAN_POINT('Origin',(-260.,-26.5,-11.5));
#56479=CARTESIAN_POINT('',(-260.,-24.7,-11.5));
#56480=CARTESIAN_POINT('Origin',(-260.,-24.7,-11.3));
#56481=CARTESIAN_POINT('Origin',(-260.,-24.7,11.3));
#57034=UNCERTAINTY_MEASURE_WITH_UNIT(LENGTH_MEASURE(0.01),#57080,
'DISTANCE_ACCURACY_VALUE',
'Maximum model space distance between geometric entities at asserted c
onnectivities');
#57040=UNCERTAINTY_MEASURE_WITH_UNIT(LENGTH_MEASURE(0.01),#57080,
'DISTANCE_ACCURACY_VALUE',
'Maximum model space distance between geometric entities at asserted c
onnectivities');
#57073=(
GEOMETRIC_REPRESENTATION_CONTEXT(3)
GLOBAL_UNCERTAINTY_ASSIGNED_CONTEXT((#57034))
GLOBAL_UNIT_ASSIGNED_CONTEXT((#57080,#57082,#57083))
REPRESENTATION_CONTEXT('','3D')
);
#57079=(
GEOMETRIC_REPRESENTATION_CONTEXT(3)
GLOBAL_UNCERTAINTY_ASSIGNED_CONTEXT((#57040))
GLOBAL_UNIT_ASSIGNED_CONTEXT((#57080,#57082,#57083))
REPRESENTATION_CONTEXT('','3D')
);
#57080=(
LENGTH_UNIT()
NAMED_UNIT(*)
SI_UNIT(.MILLI.,.METRE.)
);
#57082=(
NAMED_UNIT(*)
PLANE_ANGLE_UNIT()
SI_UNIT($,.RADIAN.)
);
#57083=(
NAMED_UNIT(*)
SI_UNIT($,.STERADIAN.)
SOLID_ANGLE_UNIT()
);
#57116=SHAPE_DEFINITION_REPRESENTATION(#57180,#57281);
#57180=PRODUCT_DEFINITION_SHAPE('',$,#57320);
#57281=SHAPE_REPRESENTATION('',(#27189),#57073);
#57287=PRODUCT_DEFINITION_CONTEXT('part definition',#57403,'design');
#57320=PRODUCT_DEFINITION('Linear Guide Spacer','Linear Guide Spacer',#57358,
#57287);
#57358=PRODUCT_DEFINITION_FORMATION('',$,#57437);
#57403=APPLICATION_CONTEXT(
'Core Data for Automotive Mechanical Design Process');
#57404=PRODUCT_CONTEXT('part definition',#57403,'mechanical');
#57437=PRODUCT('Linear Guide Spacer','Linear Guide Spacer',$,(#57404));
#57444=PRESENTATION_STYLE_ASSIGNMENT((#57446));
#57446=SURFACE_STYLE_USAGE(.BOTH.,#57448);
#57448=SURFACE_SIDE_STYLE('',(#57450));
#57450=SURFACE_STYLE_FILL_AREA(#57452);
#57452=FILL_AREA_STYLE('Opaque(202,209,238)',(#57454));
#57454=FILL_AREA_STYLE_COLOUR('Opaque(202,209,238)',#57456);
#57456=COLOUR_RGB('Opaque(202,209,238)',0.792156862745098,0.819607843137255,
0.933333333333333);
ENDSEC;
END-ISO-10303-21;
